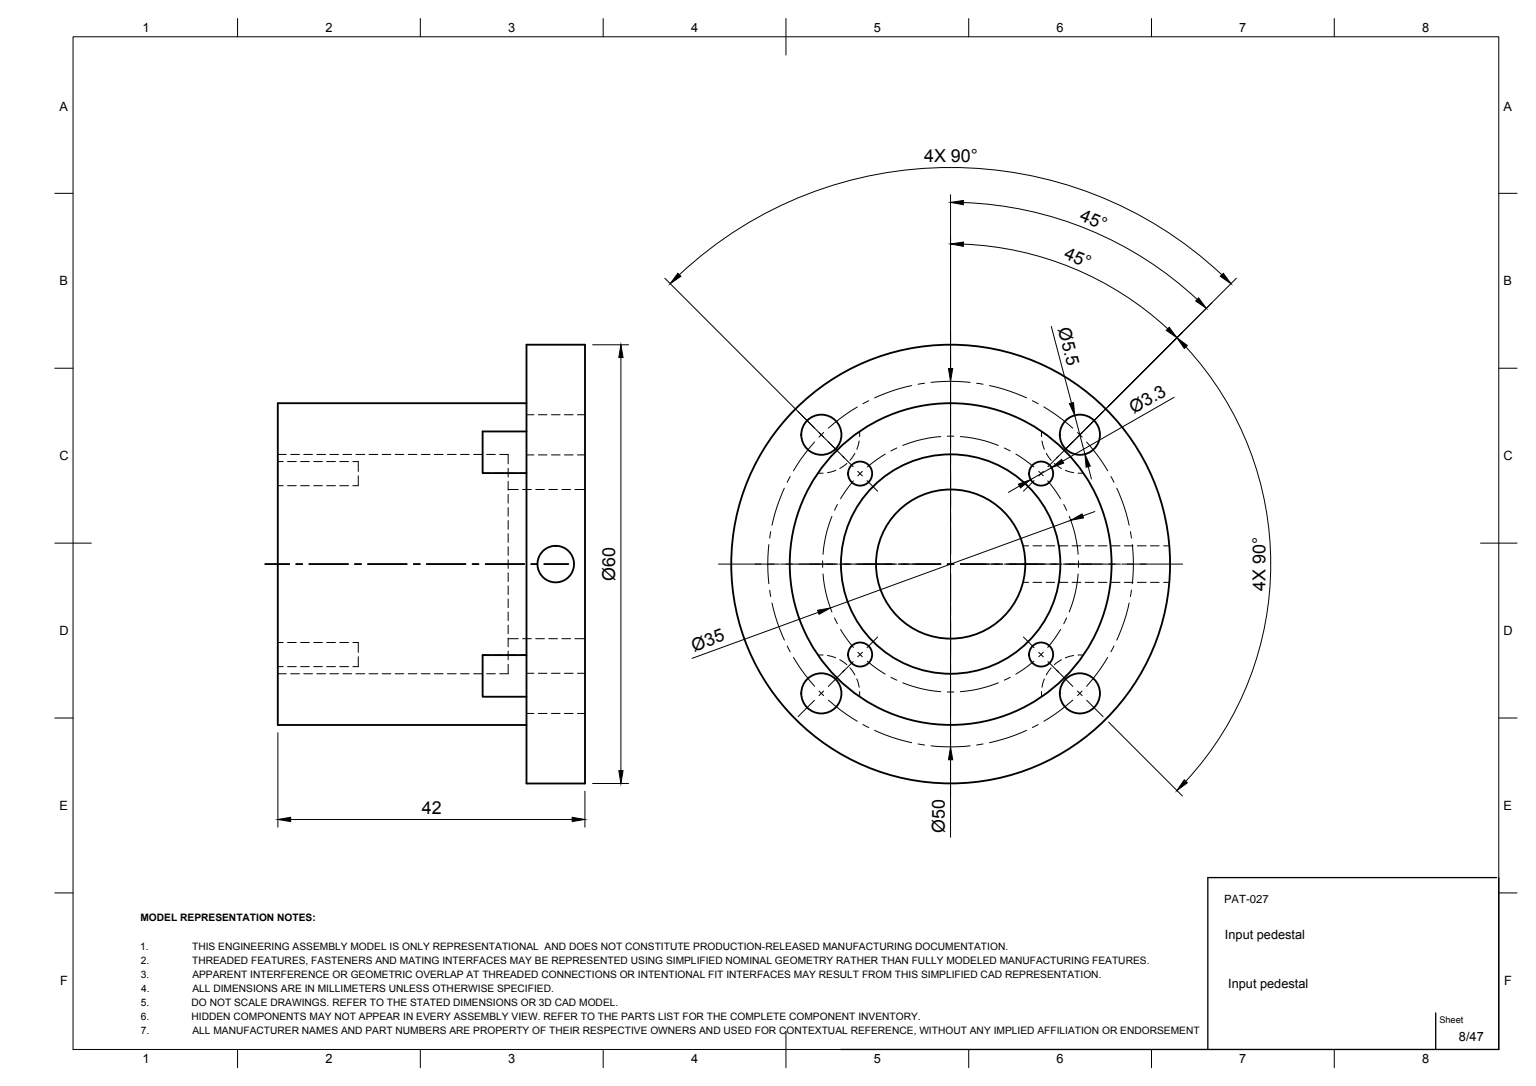
ISO-10303-21;
HEADER;
/* Generated by software containing ST-Developer
 * from STEP Tools, Inc. (www.steptools.com) 
 */

FILE_DESCRIPTION(
/* description */ ('Crank-driven oscillating fan base (mechanism only)'),

/* implementation_level */ '2;1');

FILE_NAME(
/* name */ 'Input pedestal.step',
/* time_stamp */ '2026-10-28T03:25:00-07:00',
/* author */ (''),
/* organization */ (''),
/* preprocessor_version */ 'ST-DEVELOPER v20.2',
/* originating_system */ 'Autodesk Translation Framework v15.17.0.0',
/* authorisation */ '');

FILE_SCHEMA (('AUTOMOTIVE_DESIGN { 1 0 10303 214 3 1 1 }'));
ENDSEC;

DATA;
#10=MECHANICAL_DESIGN_GEOMETRIC_PRESENTATION_REPRESENTATION('',(#440),#11916);
#316=B_SPLINE_CURVE_WITH_KNOTS('',3,(#9676,#9677,#9678,#9679,#9680,#9681,
#9682,#9683,#9684,#9685),.UNSPECIFIED.,.F.,.F.,(4,2,2,2,4),(0.,0.0945941824764479,
0.189188364952896,0.283770357603024,0.378352350253152),.UNSPECIFIED.);
#317=B_SPLINE_CURVE_WITH_KNOTS('',3,(#9686,#9687,#9688,#9689,#9690,#9691,
#9692,#9693,#9694,#9695,#9696,#9697,#9698,#9699,#9700,#9701,#9702,#9703,
#9704,#9705,#9706,#9707,#9708,#9709,#9710,#9711),.UNSPECIFIED.,.F.,.F.,
(4,2,2,2,2,2,2,2,2,2,2,2,4),(0.378352350253152,0.47293434290328,0.567516335553408,
0.662110518029855,0.756704700506303,0.851298882982751,0.945893065459199,
1.04047505810933,1.13505705075946,1.22963904340958,1.32422103605971,1.41881521853616,
1.51340940101261),.UNSPECIFIED.);
#318=B_SPLINE_CURVE_WITH_KNOTS('',3,(#9715,#9716,#9717,#9718,#9719,#9720,
#9721,#9722,#9723,#9724,#9725,#9726,#9727,#9728,#9729,#9730,#9731,#9732,
#9733,#9734,#9735,#9736,#9737,#9738,#9739,#9740),.UNSPECIFIED.,.F.,.F.,
(4,2,2,2,2,2,2,2,2,2,2,2,4),(0.,0.0942186410044058,0.188437282008812,0.282655768798837,
0.376874255588861,0.471092742378886,0.565311229168911,0.659529870173317,
0.753748511177723,0.847967152182129,0.942185793186535,1.03640427997656,
1.13062276676658),.UNSPECIFIED.);
#319=B_SPLINE_CURVE_WITH_KNOTS('',3,(#9741,#9742,#9743,#9744,#9745,#9746,
#9747,#9748,#9749,#9750),.UNSPECIFIED.,.F.,.F.,(4,2,2,2,4),(1.13062276676658,
1.22484125355661,1.31905974034663,1.41327838135104,1.50749702235545),
 .UNSPECIFIED.);
#360=SHAPE_REPRESENTATION_RELATIONSHIP('SRR','None',#12084,#400);
#400=ADVANCED_BREP_SHAPE_REPRESENTATION('',(#488),#11875);
#440=STYLED_ITEM('',(#12389),#488);
#488=MANIFOLD_SOLID_BREP('Body1',#6070);
#546=FACE_BOUND('',#1313,.T.);
#547=FACE_BOUND('',#1314,.T.);
#548=FACE_BOUND('',#1315,.T.);
#549=FACE_BOUND('',#1316,.T.);
#550=FACE_BOUND('',#1317,.T.);
#551=FACE_BOUND('',#1333,.T.);
#552=FACE_BOUND('',#1335,.T.);
#553=FACE_BOUND('',#1337,.T.);
#554=FACE_BOUND('',#1339,.T.);
#555=FACE_BOUND('',#1340,.T.);
#556=FACE_BOUND('',#1341,.T.);
#557=FACE_BOUND('',#1342,.T.);
#558=FACE_BOUND('',#1343,.T.);
#559=FACE_BOUND('',#1345,.T.);
#560=FACE_BOUND('',#1346,.T.);
#561=FACE_BOUND('',#1347,.T.);
#562=FACE_BOUND('',#1348,.T.);
#563=FACE_BOUND('',#1349,.T.);
#710=PLANE('',#6607);
#711=PLANE('',#6615);
#712=PLANE('',#6620);
#713=PLANE('',#6625);
#714=PLANE('',#6634);
#715=PLANE('',#6643);
#716=PLANE('',#6647);
#717=PLANE('',#6651);
#718=PLANE('',#6655);
#719=PLANE('',#6668);
#720=PLANE('',#6674);
#721=PLANE('',#6675);
#912=FACE_OUTER_BOUND('',#1303,.T.);
#913=FACE_OUTER_BOUND('',#1304,.T.);
#914=FACE_OUTER_BOUND('',#1305,.T.);
#915=FACE_OUTER_BOUND('',#1306,.T.);
#916=FACE_OUTER_BOUND('',#1307,.T.);
#917=FACE_OUTER_BOUND('',#1308,.T.);
#918=FACE_OUTER_BOUND('',#1309,.T.);
#919=FACE_OUTER_BOUND('',#1310,.T.);
#920=FACE_OUTER_BOUND('',#1311,.T.);
#921=FACE_OUTER_BOUND('',#1312,.T.);
#922=FACE_OUTER_BOUND('',#1318,.T.);
#923=FACE_OUTER_BOUND('',#1319,.T.);
#924=FACE_OUTER_BOUND('',#1320,.T.);
#925=FACE_OUTER_BOUND('',#1321,.T.);
#926=FACE_OUTER_BOUND('',#1322,.T.);
#927=FACE_OUTER_BOUND('',#1323,.T.);
#928=FACE_OUTER_BOUND('',#1324,.T.);
#929=FACE_OUTER_BOUND('',#1325,.T.);
#930=FACE_OUTER_BOUND('',#1326,.T.);
#931=FACE_OUTER_BOUND('',#1327,.T.);
#932=FACE_OUTER_BOUND('',#1328,.T.);
#933=FACE_OUTER_BOUND('',#1329,.T.);
#934=FACE_OUTER_BOUND('',#1330,.T.);
#935=FACE_OUTER_BOUND('',#1331,.T.);
#936=FACE_OUTER_BOUND('',#1332,.T.);
#937=FACE_OUTER_BOUND('',#1334,.T.);
#938=FACE_OUTER_BOUND('',#1336,.T.);
#939=FACE_OUTER_BOUND('',#1338,.T.);
#940=FACE_OUTER_BOUND('',#1344,.T.);
#1303=EDGE_LOOP('',(#4188,#4189));
#1304=EDGE_LOOP('',(#4190,#4191,#4192,#4193));
#1305=EDGE_LOOP('',(#4194,#4195,#4196,#4197));
#1306=EDGE_LOOP('',(#4198,#4199));
#1307=EDGE_LOOP('',(#4200,#4201,#4202,#4203));
#1308=EDGE_LOOP('',(#4204,#4205));
#1309=EDGE_LOOP('',(#4206,#4207,#4208,#4209));
#1310=EDGE_LOOP('',(#4210,#4211));
#1311=EDGE_LOOP('',(#4212,#4213,#4214,#4215,#4216,#4217,#4218,#4219,#4220,
#4221,#4222,#4223,#4224,#4225,#4226,#4227,#4228,#4229,#4230,#4231));
#1312=EDGE_LOOP('',(#4232));
#1313=EDGE_LOOP('',(#4233,#4234,#4235,#4236,#4237,#4238,#4239,#4240,#4241));
#1314=EDGE_LOOP('',(#4242));
#1315=EDGE_LOOP('',(#4243));
#1316=EDGE_LOOP('',(#4244));
#1317=EDGE_LOOP('',(#4245));
#1318=EDGE_LOOP('',(#4246,#4247,#4248,#4249));
#1319=EDGE_LOOP('',(#4250));
#1320=EDGE_LOOP('',(#4251,#4252,#4253,#4254));
#1321=EDGE_LOOP('',(#4255));
#1322=EDGE_LOOP('',(#4256,#4257,#4258,#4259));
#1323=EDGE_LOOP('',(#4260));
#1324=EDGE_LOOP('',(#4261,#4262,#4263,#4264));
#1325=EDGE_LOOP('',(#4265));
#1326=EDGE_LOOP('',(#4266,#4267,#4268,#4269,#4270,#4271));
#1327=EDGE_LOOP('',(#4272,#4273,#4274,#4275));
#1328=EDGE_LOOP('',(#4276,#4277,#4278,#4279));
#1329=EDGE_LOOP('',(#4280,#4281,#4282,#4283));
#1330=EDGE_LOOP('',(#4284,#4285,#4286,#4287));
#1331=EDGE_LOOP('',(#4288,#4289,#4290,#4291));
#1332=EDGE_LOOP('',(#4292));
#1333=EDGE_LOOP('',(#4293));
#1334=EDGE_LOOP('',(#4294,#4295,#4296,#4297));
#1335=EDGE_LOOP('',(#4298,#4299));
#1336=EDGE_LOOP('',(#4300,#4301,#4302,#4303));
#1337=EDGE_LOOP('',(#4304,#4305));
#1338=EDGE_LOOP('',(#4306));
#1339=EDGE_LOOP('',(#4307));
#1340=EDGE_LOOP('',(#4308));
#1341=EDGE_LOOP('',(#4309));
#1342=EDGE_LOOP('',(#4310));
#1343=EDGE_LOOP('',(#4311));
#1344=EDGE_LOOP('',(#4312));
#1345=EDGE_LOOP('',(#4313));
#1346=EDGE_LOOP('',(#4314));
#1347=EDGE_LOOP('',(#4315));
#1348=EDGE_LOOP('',(#4316));
#1349=EDGE_LOOP('',(#4317));
#1842=LINE('',#9587,#2175);
#1843=LINE('',#9590,#2176);
#1844=LINE('',#9594,#2177);
#1845=LINE('',#9598,#2178);
#1846=LINE('',#9605,#2179);
#1847=LINE('',#9609,#2180);
#1848=LINE('',#9616,#2181);
#1849=LINE('',#9620,#2182);
#1850=LINE('',#9628,#2183);
#1851=LINE('',#9649,#2184);
#1852=LINE('',#9656,#2185);
#1853=LINE('',#9663,#2186);
#1854=LINE('',#9670,#2187);
#1855=LINE('',#9713,#2188);
#1856=LINE('',#9754,#2189);
#1857=LINE('',#9758,#2190);
#1858=LINE('',#9762,#2191);
#1859=LINE('',#9766,#2192);
#1860=LINE('',#9771,#2193);
#1861=LINE('',#9778,#2194);
#1862=LINE('',#9782,#2195);
#2175=VECTOR('',#7559,1.);
#2176=VECTOR('',#7562,1.);
#2177=VECTOR('',#7565,1.);
#2178=VECTOR('',#7568,1.);
#2179=VECTOR('',#7577,1.);
#2180=VECTOR('',#7580,1.);
#2181=VECTOR('',#7589,1.);
#2182=VECTOR('',#7592,1.);
#2183=VECTOR('',#7603,2.2);
#2184=VECTOR('',#7630,0.165);
#2185=VECTOR('',#7639,0.165);
#2186=VECTOR('',#7648,0.165);
#2187=VECTOR('',#7657,0.165);
#2188=VECTOR('',#7664,0.25);
#2189=VECTOR('',#7669,0.275);
#2190=VECTOR('',#7674,0.275);
#2191=VECTOR('',#7679,0.275);
#2192=VECTOR('',#7684,0.275);
#2193=VECTOR('',#7689,1.5);
#2194=VECTOR('',#7698,3.);
#2195=VECTOR('',#7703,1.02);
#2480=CIRCLE('',#6608,2.2);
#2481=CIRCLE('',#6609,0.525);
#2482=CIRCLE('',#6611,0.525);
#2483=CIRCLE('',#6613,0.525);
#2484=CIRCLE('',#6614,0.525);
#2485=CIRCLE('',#6616,2.2);
#2486=CIRCLE('',#6618,0.525);
#2487=CIRCLE('',#6619,0.525);
#2488=CIRCLE('',#6621,2.2);
#2489=CIRCLE('',#6623,0.525);
#2490=CIRCLE('',#6624,0.525);
#2491=CIRCLE('',#6626,2.2);
#2492=CIRCLE('',#6628,2.2);
#2493=CIRCLE('',#6629,2.2);
#2494=CIRCLE('',#6630,2.2);
#2495=CIRCLE('',#6631,2.2);
#2496=CIRCLE('',#6632,2.2);
#2497=CIRCLE('',#6633,2.2);
#2498=CIRCLE('',#6635,3.);
#2499=CIRCLE('',#6636,0.275);
#2500=CIRCLE('',#6637,0.275);
#2501=CIRCLE('',#6638,0.275);
#2502=CIRCLE('',#6639,0.275);
#2503=CIRCLE('',#6641,0.165);
#2504=CIRCLE('',#6642,0.165);
#2505=CIRCLE('',#6645,0.165);
#2506=CIRCLE('',#6646,0.165);
#2507=CIRCLE('',#6649,0.165);
#2508=CIRCLE('',#6650,0.165);
#2509=CIRCLE('',#6653,0.165);
#2510=CIRCLE('',#6654,0.165);
#2511=CIRCLE('',#6658,0.275);
#2512=CIRCLE('',#6660,0.275);
#2513=CIRCLE('',#6662,0.275);
#2514=CIRCLE('',#6664,0.275);
#2515=CIRCLE('',#6666,1.5);
#2516=CIRCLE('',#6667,1.5);
#2517=CIRCLE('',#6669,1.02);
#2518=CIRCLE('',#6671,3.);
#2519=CIRCLE('',#6673,1.02);
#2869=VERTEX_POINT('',#9581);
#2870=VERTEX_POINT('',#9582);
#2871=VERTEX_POINT('',#9586);
#2872=VERTEX_POINT('',#9588);
#2873=VERTEX_POINT('',#9592);
#2874=VERTEX_POINT('',#9593);
#2875=VERTEX_POINT('',#9595);
#2876=VERTEX_POINT('',#9597);
#2877=VERTEX_POINT('',#9603);
#2878=VERTEX_POINT('',#9604);
#2879=VERTEX_POINT('',#9606);
#2880=VERTEX_POINT('',#9608);
#2881=VERTEX_POINT('',#9614);
#2882=VERTEX_POINT('',#9615);
#2883=VERTEX_POINT('',#9617);
#2884=VERTEX_POINT('',#9619);
#2885=VERTEX_POINT('',#9625);
#2886=VERTEX_POINT('',#9627);
#2887=VERTEX_POINT('',#9635);
#2888=VERTEX_POINT('',#9637);
#2889=VERTEX_POINT('',#9639);
#2890=VERTEX_POINT('',#9641);
#2891=VERTEX_POINT('',#9643);
#2892=VERTEX_POINT('',#9646);
#2893=VERTEX_POINT('',#9648);
#2894=VERTEX_POINT('',#9653);
#2895=VERTEX_POINT('',#9655);
#2896=VERTEX_POINT('',#9660);
#2897=VERTEX_POINT('',#9662);
#2898=VERTEX_POINT('',#9667);
#2899=VERTEX_POINT('',#9669);
#2900=VERTEX_POINT('',#9674);
#2901=VERTEX_POINT('',#9675);
#2902=VERTEX_POINT('',#9712);
#2903=VERTEX_POINT('',#9714);
#2904=VERTEX_POINT('',#9752);
#2905=VERTEX_POINT('',#9756);
#2906=VERTEX_POINT('',#9760);
#2907=VERTEX_POINT('',#9764);
#2908=VERTEX_POINT('',#9768);
#2909=VERTEX_POINT('',#9770);
#2910=VERTEX_POINT('',#9774);
#2911=VERTEX_POINT('',#9777);
#2912=VERTEX_POINT('',#9781);
#3389=EDGE_CURVE('',#2869,#2870,#2480,.T.);
#3390=EDGE_CURVE('',#2870,#2869,#2481,.T.);
#3391=EDGE_CURVE('',#2871,#2869,#1842,.T.);
#3392=EDGE_CURVE('',#2872,#2871,#2482,.T.);
#3393=EDGE_CURVE('',#2870,#2872,#1843,.T.);
#3394=EDGE_CURVE('',#2873,#2874,#1844,.T.);
#3395=EDGE_CURVE('',#2873,#2875,#2483,.T.);
#3396=EDGE_CURVE('',#2876,#2875,#1845,.T.);
#3397=EDGE_CURVE('',#2874,#2876,#2484,.T.);
#3398=EDGE_CURVE('',#2875,#2873,#2485,.T.);
#3399=EDGE_CURVE('',#2877,#2878,#1846,.T.);
#3400=EDGE_CURVE('',#2877,#2879,#2486,.T.);
#3401=EDGE_CURVE('',#2880,#2879,#1847,.T.);
#3402=EDGE_CURVE('',#2878,#2880,#2487,.T.);
#3403=EDGE_CURVE('',#2879,#2877,#2488,.T.);
#3404=EDGE_CURVE('',#2881,#2882,#1848,.T.);
#3405=EDGE_CURVE('',#2881,#2883,#2489,.T.);
#3406=EDGE_CURVE('',#2884,#2883,#1849,.T.);
#3407=EDGE_CURVE('',#2882,#2884,#2490,.T.);
#3408=EDGE_CURVE('',#2883,#2881,#2491,.T.);
#3409=EDGE_CURVE('',#2885,#2885,#2492,.T.);
#3410=EDGE_CURVE('',#2885,#2886,#1850,.T.);
#3411=EDGE_CURVE('',#2886,#2871,#2493,.T.);
#3412=EDGE_CURVE('',#2872,#2884,#2494,.T.);
#3413=EDGE_CURVE('',#2882,#2880,#2495,.T.);
#3414=EDGE_CURVE('',#2878,#2876,#2496,.T.);
#3415=EDGE_CURVE('',#2874,#2886,#2497,.T.);
#3416=EDGE_CURVE('',#2887,#2887,#2498,.T.);
#3417=EDGE_CURVE('',#2888,#2888,#2499,.T.);
#3418=EDGE_CURVE('',#2889,#2889,#2500,.T.);
#3419=EDGE_CURVE('',#2890,#2890,#2501,.T.);
#3420=EDGE_CURVE('',#2891,#2891,#2502,.T.);
#3421=EDGE_CURVE('',#2892,#2892,#2503,.T.);
#3422=EDGE_CURVE('',#2892,#2893,#1851,.T.);
#3423=EDGE_CURVE('',#2893,#2893,#2504,.T.);
#3424=EDGE_CURVE('',#2894,#2894,#2505,.T.);
#3425=EDGE_CURVE('',#2894,#2895,#1852,.T.);
#3426=EDGE_CURVE('',#2895,#2895,#2506,.T.);
#3427=EDGE_CURVE('',#2896,#2896,#2507,.T.);
#3428=EDGE_CURVE('',#2896,#2897,#1853,.T.);
#3429=EDGE_CURVE('',#2897,#2897,#2508,.T.);
#3430=EDGE_CURVE('',#2898,#2898,#2509,.T.);
#3431=EDGE_CURVE('',#2898,#2899,#1854,.T.);
#3432=EDGE_CURVE('',#2899,#2899,#2510,.T.);
#3433=EDGE_CURVE('',#2900,#2901,#316,.T.);
#3434=EDGE_CURVE('',#2901,#2900,#317,.T.);
#3435=EDGE_CURVE('',#2901,#2902,#1855,.T.);
#3436=EDGE_CURVE('',#2903,#2902,#318,.T.);
#3437=EDGE_CURVE('',#2902,#2903,#319,.T.);
#3438=EDGE_CURVE('',#2904,#2904,#2511,.T.);
#3439=EDGE_CURVE('',#2904,#2888,#1856,.T.);
#3440=EDGE_CURVE('',#2905,#2905,#2512,.T.);
#3441=EDGE_CURVE('',#2905,#2891,#1857,.T.);
#3442=EDGE_CURVE('',#2906,#2906,#2513,.T.);
#3443=EDGE_CURVE('',#2906,#2889,#1858,.T.);
#3444=EDGE_CURVE('',#2907,#2907,#2514,.T.);
#3445=EDGE_CURVE('',#2907,#2890,#1859,.T.);
#3446=EDGE_CURVE('',#2908,#2908,#2515,.T.);
#3447=EDGE_CURVE('',#2908,#2909,#1860,.T.);
#3448=EDGE_CURVE('',#2909,#2909,#2516,.T.);
#3449=EDGE_CURVE('',#2910,#2910,#2517,.T.);
#3450=EDGE_CURVE('',#2887,#2911,#1861,.T.);
#3451=EDGE_CURVE('',#2911,#2911,#2518,.T.);
#3452=EDGE_CURVE('',#2910,#2912,#1862,.T.);
#3453=EDGE_CURVE('',#2912,#2912,#2519,.T.);
#4188=ORIENTED_EDGE('',*,*,#3389,.F.);
#4189=ORIENTED_EDGE('',*,*,#3390,.F.);
#4190=ORIENTED_EDGE('',*,*,#3391,.F.);
#4191=ORIENTED_EDGE('',*,*,#3392,.F.);
#4192=ORIENTED_EDGE('',*,*,#3393,.F.);
#4193=ORIENTED_EDGE('',*,*,#3390,.T.);
#4194=ORIENTED_EDGE('',*,*,#3394,.F.);
#4195=ORIENTED_EDGE('',*,*,#3395,.T.);
#4196=ORIENTED_EDGE('',*,*,#3396,.F.);
#4197=ORIENTED_EDGE('',*,*,#3397,.F.);
#4198=ORIENTED_EDGE('',*,*,#3398,.F.);
#4199=ORIENTED_EDGE('',*,*,#3395,.F.);
#4200=ORIENTED_EDGE('',*,*,#3399,.F.);
#4201=ORIENTED_EDGE('',*,*,#3400,.T.);
#4202=ORIENTED_EDGE('',*,*,#3401,.F.);
#4203=ORIENTED_EDGE('',*,*,#3402,.F.);
#4204=ORIENTED_EDGE('',*,*,#3403,.F.);
#4205=ORIENTED_EDGE('',*,*,#3400,.F.);
#4206=ORIENTED_EDGE('',*,*,#3404,.F.);
#4207=ORIENTED_EDGE('',*,*,#3405,.T.);
#4208=ORIENTED_EDGE('',*,*,#3406,.F.);
#4209=ORIENTED_EDGE('',*,*,#3407,.F.);
#4210=ORIENTED_EDGE('',*,*,#3408,.F.);
#4211=ORIENTED_EDGE('',*,*,#3405,.F.);
#4212=ORIENTED_EDGE('',*,*,#3409,.F.);
#4213=ORIENTED_EDGE('',*,*,#3410,.T.);
#4214=ORIENTED_EDGE('',*,*,#3411,.T.);
#4215=ORIENTED_EDGE('',*,*,#3391,.T.);
#4216=ORIENTED_EDGE('',*,*,#3389,.T.);
#4217=ORIENTED_EDGE('',*,*,#3393,.T.);
#4218=ORIENTED_EDGE('',*,*,#3412,.T.);
#4219=ORIENTED_EDGE('',*,*,#3406,.T.);
#4220=ORIENTED_EDGE('',*,*,#3408,.T.);
#4221=ORIENTED_EDGE('',*,*,#3404,.T.);
#4222=ORIENTED_EDGE('',*,*,#3413,.T.);
#4223=ORIENTED_EDGE('',*,*,#3401,.T.);
#4224=ORIENTED_EDGE('',*,*,#3403,.T.);
#4225=ORIENTED_EDGE('',*,*,#3399,.T.);
#4226=ORIENTED_EDGE('',*,*,#3414,.T.);
#4227=ORIENTED_EDGE('',*,*,#3396,.T.);
#4228=ORIENTED_EDGE('',*,*,#3398,.T.);
#4229=ORIENTED_EDGE('',*,*,#3394,.T.);
#4230=ORIENTED_EDGE('',*,*,#3415,.T.);
#4231=ORIENTED_EDGE('',*,*,#3410,.F.);
#4232=ORIENTED_EDGE('',*,*,#3416,.T.);
#4233=ORIENTED_EDGE('',*,*,#3415,.F.);
#4234=ORIENTED_EDGE('',*,*,#3397,.T.);
#4235=ORIENTED_EDGE('',*,*,#3414,.F.);
#4236=ORIENTED_EDGE('',*,*,#3402,.T.);
#4237=ORIENTED_EDGE('',*,*,#3413,.F.);
#4238=ORIENTED_EDGE('',*,*,#3407,.T.);
#4239=ORIENTED_EDGE('',*,*,#3412,.F.);
#4240=ORIENTED_EDGE('',*,*,#3392,.T.);
#4241=ORIENTED_EDGE('',*,*,#3411,.F.);
#4242=ORIENTED_EDGE('',*,*,#3417,.T.);
#4243=ORIENTED_EDGE('',*,*,#3418,.T.);
#4244=ORIENTED_EDGE('',*,*,#3419,.T.);
#4245=ORIENTED_EDGE('',*,*,#3420,.T.);
#4246=ORIENTED_EDGE('',*,*,#3421,.F.);
#4247=ORIENTED_EDGE('',*,*,#3422,.T.);
#4248=ORIENTED_EDGE('',*,*,#3423,.F.);
#4249=ORIENTED_EDGE('',*,*,#3422,.F.);
#4250=ORIENTED_EDGE('',*,*,#3421,.T.);
#4251=ORIENTED_EDGE('',*,*,#3424,.F.);
#4252=ORIENTED_EDGE('',*,*,#3425,.T.);
#4253=ORIENTED_EDGE('',*,*,#3426,.F.);
#4254=ORIENTED_EDGE('',*,*,#3425,.F.);
#4255=ORIENTED_EDGE('',*,*,#3424,.T.);
#4256=ORIENTED_EDGE('',*,*,#3427,.F.);
#4257=ORIENTED_EDGE('',*,*,#3428,.T.);
#4258=ORIENTED_EDGE('',*,*,#3429,.F.);
#4259=ORIENTED_EDGE('',*,*,#3428,.F.);
#4260=ORIENTED_EDGE('',*,*,#3427,.T.);
#4261=ORIENTED_EDGE('',*,*,#3430,.F.);
#4262=ORIENTED_EDGE('',*,*,#3431,.T.);
#4263=ORIENTED_EDGE('',*,*,#3432,.F.);
#4264=ORIENTED_EDGE('',*,*,#3431,.F.);
#4265=ORIENTED_EDGE('',*,*,#3430,.T.);
#4266=ORIENTED_EDGE('',*,*,#3433,.F.);
#4267=ORIENTED_EDGE('',*,*,#3434,.F.);
#4268=ORIENTED_EDGE('',*,*,#3435,.T.);
#4269=ORIENTED_EDGE('',*,*,#3436,.F.);
#4270=ORIENTED_EDGE('',*,*,#3437,.F.);
#4271=ORIENTED_EDGE('',*,*,#3435,.F.);
#4272=ORIENTED_EDGE('',*,*,#3438,.F.);
#4273=ORIENTED_EDGE('',*,*,#3439,.T.);
#4274=ORIENTED_EDGE('',*,*,#3417,.F.);
#4275=ORIENTED_EDGE('',*,*,#3439,.F.);
#4276=ORIENTED_EDGE('',*,*,#3440,.F.);
#4277=ORIENTED_EDGE('',*,*,#3441,.T.);
#4278=ORIENTED_EDGE('',*,*,#3420,.F.);
#4279=ORIENTED_EDGE('',*,*,#3441,.F.);
#4280=ORIENTED_EDGE('',*,*,#3442,.F.);
#4281=ORIENTED_EDGE('',*,*,#3443,.T.);
#4282=ORIENTED_EDGE('',*,*,#3418,.F.);
#4283=ORIENTED_EDGE('',*,*,#3443,.F.);
#4284=ORIENTED_EDGE('',*,*,#3444,.F.);
#4285=ORIENTED_EDGE('',*,*,#3445,.T.);
#4286=ORIENTED_EDGE('',*,*,#3419,.F.);
#4287=ORIENTED_EDGE('',*,*,#3445,.F.);
#4288=ORIENTED_EDGE('',*,*,#3446,.F.);
#4289=ORIENTED_EDGE('',*,*,#3447,.T.);
#4290=ORIENTED_EDGE('',*,*,#3448,.F.);
#4291=ORIENTED_EDGE('',*,*,#3447,.F.);
#4292=ORIENTED_EDGE('',*,*,#3446,.T.);
#4293=ORIENTED_EDGE('',*,*,#3449,.F.);
#4294=ORIENTED_EDGE('',*,*,#3416,.F.);
#4295=ORIENTED_EDGE('',*,*,#3450,.T.);
#4296=ORIENTED_EDGE('',*,*,#3451,.T.);
#4297=ORIENTED_EDGE('',*,*,#3450,.F.);
#4298=ORIENTED_EDGE('',*,*,#3436,.T.);
#4299=ORIENTED_EDGE('',*,*,#3437,.T.);
#4300=ORIENTED_EDGE('',*,*,#3449,.T.);
#4301=ORIENTED_EDGE('',*,*,#3452,.T.);
#4302=ORIENTED_EDGE('',*,*,#3453,.T.);
#4303=ORIENTED_EDGE('',*,*,#3452,.F.);
#4304=ORIENTED_EDGE('',*,*,#3433,.T.);
#4305=ORIENTED_EDGE('',*,*,#3434,.T.);
#4306=ORIENTED_EDGE('',*,*,#3409,.T.);
#4307=ORIENTED_EDGE('',*,*,#3448,.T.);
#4308=ORIENTED_EDGE('',*,*,#3432,.T.);
#4309=ORIENTED_EDGE('',*,*,#3429,.T.);
#4310=ORIENTED_EDGE('',*,*,#3426,.T.);
#4311=ORIENTED_EDGE('',*,*,#3423,.T.);
#4312=ORIENTED_EDGE('',*,*,#3451,.F.);
#4313=ORIENTED_EDGE('',*,*,#3453,.F.);
#4314=ORIENTED_EDGE('',*,*,#3444,.T.);
#4315=ORIENTED_EDGE('',*,*,#3442,.T.);
#4316=ORIENTED_EDGE('',*,*,#3440,.T.);
#4317=ORIENTED_EDGE('',*,*,#3438,.T.);
#5554=CYLINDRICAL_SURFACE('',#6610,0.525);
#5555=CYLINDRICAL_SURFACE('',#6612,0.525);
#5556=CYLINDRICAL_SURFACE('',#6617,0.525);
#5557=CYLINDRICAL_SURFACE('',#6622,0.525);
#5558=CYLINDRICAL_SURFACE('',#6627,2.2);
#5559=CYLINDRICAL_SURFACE('',#6640,0.165);
#5560=CYLINDRICAL_SURFACE('',#6644,0.165);
#5561=CYLINDRICAL_SURFACE('',#6648,0.165);
#5562=CYLINDRICAL_SURFACE('',#6652,0.165);
#5563=CYLINDRICAL_SURFACE('',#6656,0.25);
#5564=CYLINDRICAL_SURFACE('',#6657,0.275);
#5565=CYLINDRICAL_SURFACE('',#6659,0.275);
#5566=CYLINDRICAL_SURFACE('',#6661,0.275);
#5567=CYLINDRICAL_SURFACE('',#6663,0.275);
#5568=CYLINDRICAL_SURFACE('',#6665,1.5);
#5569=CYLINDRICAL_SURFACE('',#6670,3.);
#5570=CYLINDRICAL_SURFACE('',#6672,1.02);
#5718=ADVANCED_FACE('',(#912),#710,.F.);
#5719=ADVANCED_FACE('',(#913),#5554,.F.);
#5720=ADVANCED_FACE('',(#914),#5555,.F.);
#5721=ADVANCED_FACE('',(#915),#711,.F.);
#5722=ADVANCED_FACE('',(#916),#5556,.F.);
#5723=ADVANCED_FACE('',(#917),#712,.F.);
#5724=ADVANCED_FACE('',(#918),#5557,.F.);
#5725=ADVANCED_FACE('',(#919),#713,.F.);
#5726=ADVANCED_FACE('',(#920),#5558,.T.);
#5727=ADVANCED_FACE('',(#921,#546,#547,#548,#549,#550),#714,.T.);
#5728=ADVANCED_FACE('',(#922),#5559,.F.);
#5729=ADVANCED_FACE('',(#923),#715,.T.);
#5730=ADVANCED_FACE('',(#924),#5560,.F.);
#5731=ADVANCED_FACE('',(#925),#716,.T.);
#5732=ADVANCED_FACE('',(#926),#5561,.F.);
#5733=ADVANCED_FACE('',(#927),#717,.T.);
#5734=ADVANCED_FACE('',(#928),#5562,.F.);
#5735=ADVANCED_FACE('',(#929),#718,.T.);
#5736=ADVANCED_FACE('',(#930),#5563,.F.);
#5737=ADVANCED_FACE('',(#931),#5564,.F.);
#5738=ADVANCED_FACE('',(#932),#5565,.F.);
#5739=ADVANCED_FACE('',(#933),#5566,.F.);
#5740=ADVANCED_FACE('',(#934),#5567,.F.);
#5741=ADVANCED_FACE('',(#935),#5568,.F.);
#5742=ADVANCED_FACE('',(#936,#551),#719,.T.);
#5743=ADVANCED_FACE('',(#937,#552),#5569,.T.);
#5744=ADVANCED_FACE('',(#938,#553),#5570,.F.);
#5745=ADVANCED_FACE('',(#939,#554,#555,#556,#557,#558),#720,.T.);
#5746=ADVANCED_FACE('',(#940,#559,#560,#561,#562,#563),#721,.F.);
#6070=CLOSED_SHELL('',(#5718,#5719,#5720,#5721,#5722,#5723,#5724,#5725,
#5726,#5727,#5728,#5729,#5730,#5731,#5732,#5733,#5734,#5735,#5736,#5737,
#5738,#5739,#5740,#5741,#5742,#5743,#5744,#5745,#5746));
#6606=AXIS2_PLACEMENT_3D('',#9579,#7549,#7550);
#6607=AXIS2_PLACEMENT_3D('',#9580,#7551,#7552);
#6608=AXIS2_PLACEMENT_3D('',#9583,#7553,#7554);
#6609=AXIS2_PLACEMENT_3D('',#9584,#7555,#7556);
#6610=AXIS2_PLACEMENT_3D('',#9585,#7557,#7558);
#6611=AXIS2_PLACEMENT_3D('',#9589,#7560,#7561);
#6612=AXIS2_PLACEMENT_3D('',#9591,#7563,#7564);
#6613=AXIS2_PLACEMENT_3D('',#9596,#7566,#7567);
#6614=AXIS2_PLACEMENT_3D('',#9599,#7569,#7570);
#6615=AXIS2_PLACEMENT_3D('',#9600,#7571,#7572);
#6616=AXIS2_PLACEMENT_3D('',#9601,#7573,#7574);
#6617=AXIS2_PLACEMENT_3D('',#9602,#7575,#7576);
#6618=AXIS2_PLACEMENT_3D('',#9607,#7578,#7579);
#6619=AXIS2_PLACEMENT_3D('',#9610,#7581,#7582);
#6620=AXIS2_PLACEMENT_3D('',#9611,#7583,#7584);
#6621=AXIS2_PLACEMENT_3D('',#9612,#7585,#7586);
#6622=AXIS2_PLACEMENT_3D('',#9613,#7587,#7588);
#6623=AXIS2_PLACEMENT_3D('',#9618,#7590,#7591);
#6624=AXIS2_PLACEMENT_3D('',#9621,#7593,#7594);
#6625=AXIS2_PLACEMENT_3D('',#9622,#7595,#7596);
#6626=AXIS2_PLACEMENT_3D('',#9623,#7597,#7598);
#6627=AXIS2_PLACEMENT_3D('',#9624,#7599,#7600);
#6628=AXIS2_PLACEMENT_3D('',#9626,#7601,#7602);
#6629=AXIS2_PLACEMENT_3D('',#9629,#7604,#7605);
#6630=AXIS2_PLACEMENT_3D('',#9630,#7606,#7607);
#6631=AXIS2_PLACEMENT_3D('',#9631,#7608,#7609);
#6632=AXIS2_PLACEMENT_3D('',#9632,#7610,#7611);
#6633=AXIS2_PLACEMENT_3D('',#9633,#7612,#7613);
#6634=AXIS2_PLACEMENT_3D('',#9634,#7614,#7615);
#6635=AXIS2_PLACEMENT_3D('',#9636,#7616,#7617);
#6636=AXIS2_PLACEMENT_3D('',#9638,#7618,#7619);
#6637=AXIS2_PLACEMENT_3D('',#9640,#7620,#7621);
#6638=AXIS2_PLACEMENT_3D('',#9642,#7622,#7623);
#6639=AXIS2_PLACEMENT_3D('',#9644,#7624,#7625);
#6640=AXIS2_PLACEMENT_3D('',#9645,#7626,#7627);
#6641=AXIS2_PLACEMENT_3D('',#9647,#7628,#7629);
#6642=AXIS2_PLACEMENT_3D('',#9650,#7631,#7632);
#6643=AXIS2_PLACEMENT_3D('',#9651,#7633,#7634);
#6644=AXIS2_PLACEMENT_3D('',#9652,#7635,#7636);
#6645=AXIS2_PLACEMENT_3D('',#9654,#7637,#7638);
#6646=AXIS2_PLACEMENT_3D('',#9657,#7640,#7641);
#6647=AXIS2_PLACEMENT_3D('',#9658,#7642,#7643);
#6648=AXIS2_PLACEMENT_3D('',#9659,#7644,#7645);
#6649=AXIS2_PLACEMENT_3D('',#9661,#7646,#7647);
#6650=AXIS2_PLACEMENT_3D('',#9664,#7649,#7650);
#6651=AXIS2_PLACEMENT_3D('',#9665,#7651,#7652);
#6652=AXIS2_PLACEMENT_3D('',#9666,#7653,#7654);
#6653=AXIS2_PLACEMENT_3D('',#9668,#7655,#7656);
#6654=AXIS2_PLACEMENT_3D('',#9671,#7658,#7659);
#6655=AXIS2_PLACEMENT_3D('',#9672,#7660,#7661);
#6656=AXIS2_PLACEMENT_3D('',#9673,#7662,#7663);
#6657=AXIS2_PLACEMENT_3D('',#9751,#7665,#7666);
#6658=AXIS2_PLACEMENT_3D('',#9753,#7667,#7668);
#6659=AXIS2_PLACEMENT_3D('',#9755,#7670,#7671);
#6660=AXIS2_PLACEMENT_3D('',#9757,#7672,#7673);
#6661=AXIS2_PLACEMENT_3D('',#9759,#7675,#7676);
#6662=AXIS2_PLACEMENT_3D('',#9761,#7677,#7678);
#6663=AXIS2_PLACEMENT_3D('',#9763,#7680,#7681);
#6664=AXIS2_PLACEMENT_3D('',#9765,#7682,#7683);
#6665=AXIS2_PLACEMENT_3D('',#9767,#7685,#7686);
#6666=AXIS2_PLACEMENT_3D('',#9769,#7687,#7688);
#6667=AXIS2_PLACEMENT_3D('',#9772,#7690,#7691);
#6668=AXIS2_PLACEMENT_3D('',#9773,#7692,#7693);
#6669=AXIS2_PLACEMENT_3D('',#9775,#7694,#7695);
#6670=AXIS2_PLACEMENT_3D('',#9776,#7696,#7697);
#6671=AXIS2_PLACEMENT_3D('',#9779,#7699,#7700);
#6672=AXIS2_PLACEMENT_3D('',#9780,#7701,#7702);
#6673=AXIS2_PLACEMENT_3D('',#9783,#7704,#7705);
#6674=AXIS2_PLACEMENT_3D('',#9784,#7706,#7707);
#6675=AXIS2_PLACEMENT_3D('',#9785,#7708,#7709);
#7549=DIRECTION('axis',(0.,0.,1.));
#7550=DIRECTION('refdir',(1.,0.,0.));
#7551=DIRECTION('center_axis',(0.,0.,1.));
#7552=DIRECTION('ref_axis',(1.,0.,0.));
#7553=DIRECTION('center_axis',(0.,0.,1.));
#7554=DIRECTION('ref_axis',(1.,0.,0.));
#7555=DIRECTION('center_axis',(0.,0.,1.));
#7556=DIRECTION('ref_axis',(1.,0.,0.));
#7557=DIRECTION('center_axis',(0.,0.,1.));
#7558=DIRECTION('ref_axis',(1.,0.,0.));
#7559=DIRECTION('',(0.,0.,1.));
#7560=DIRECTION('center_axis',(0.,0.,1.));
#7561=DIRECTION('ref_axis',(1.,0.,0.));
#7562=DIRECTION('',(0.,0.,-1.));
#7563=DIRECTION('center_axis',(0.,0.,1.));
#7564=DIRECTION('ref_axis',(1.,0.,0.));
#7565=DIRECTION('',(0.,0.,-1.));
#7566=DIRECTION('center_axis',(0.,0.,1.));
#7567=DIRECTION('ref_axis',(1.,0.,0.));
#7568=DIRECTION('',(0.,0.,1.));
#7569=DIRECTION('center_axis',(0.,0.,1.));
#7570=DIRECTION('ref_axis',(1.,0.,0.));
#7571=DIRECTION('center_axis',(0.,0.,1.));
#7572=DIRECTION('ref_axis',(1.,0.,0.));
#7573=DIRECTION('center_axis',(0.,0.,1.));
#7574=DIRECTION('ref_axis',(1.,0.,0.));
#7575=DIRECTION('center_axis',(0.,0.,1.));
#7576=DIRECTION('ref_axis',(-0.707106781186548,-0.707106781186547,0.));
#7577=DIRECTION('',(0.,0.,-1.));
#7578=DIRECTION('center_axis',(0.,0.,1.));
#7579=DIRECTION('ref_axis',(1.,0.,0.));
#7580=DIRECTION('',(0.,0.,1.));
#7581=DIRECTION('center_axis',(0.,0.,1.));
#7582=DIRECTION('ref_axis',(1.,0.,0.));
#7583=DIRECTION('center_axis',(0.,0.,1.));
#7584=DIRECTION('ref_axis',(1.,0.,0.));
#7585=DIRECTION('center_axis',(0.,0.,1.));
#7586=DIRECTION('ref_axis',(1.,0.,0.));
#7587=DIRECTION('center_axis',(0.,0.,1.));
#7588=DIRECTION('ref_axis',(-0.707106781186547,0.707106781186548,0.));
#7589=DIRECTION('',(0.,0.,-1.));
#7590=DIRECTION('center_axis',(0.,0.,1.));
#7591=DIRECTION('ref_axis',(1.,0.,0.));
#7592=DIRECTION('',(0.,0.,1.));
#7593=DIRECTION('center_axis',(0.,0.,1.));
#7594=DIRECTION('ref_axis',(1.,0.,0.));
#7595=DIRECTION('center_axis',(0.,0.,1.));
#7596=DIRECTION('ref_axis',(1.,0.,0.));
#7597=DIRECTION('center_axis',(0.,0.,1.));
#7598=DIRECTION('ref_axis',(1.,0.,0.));
#7599=DIRECTION('center_axis',(0.,0.,1.));
#7600=DIRECTION('ref_axis',(1.,0.,0.));
#7601=DIRECTION('center_axis',(0.,0.,1.));
#7602=DIRECTION('ref_axis',(1.,0.,0.));
#7603=DIRECTION('',(0.,0.,-1.));
#7604=DIRECTION('center_axis',(0.,0.,1.));
#7605=DIRECTION('ref_axis',(1.,0.,0.));
#7606=DIRECTION('center_axis',(0.,0.,1.));
#7607=DIRECTION('ref_axis',(1.,0.,0.));
#7608=DIRECTION('center_axis',(0.,0.,1.));
#7609=DIRECTION('ref_axis',(1.,0.,0.));
#7610=DIRECTION('center_axis',(0.,0.,1.));
#7611=DIRECTION('ref_axis',(1.,0.,0.));
#7612=DIRECTION('center_axis',(0.,0.,1.));
#7613=DIRECTION('ref_axis',(1.,0.,0.));
#7614=DIRECTION('center_axis',(0.,0.,1.));
#7615=DIRECTION('ref_axis',(1.,0.,0.));
#7616=DIRECTION('center_axis',(0.,0.,1.));
#7617=DIRECTION('ref_axis',(1.,0.,0.));
#7618=DIRECTION('center_axis',(0.,0.,-1.));
#7619=DIRECTION('ref_axis',(1.,0.,0.));
#7620=DIRECTION('center_axis',(0.,0.,-1.));
#7621=DIRECTION('ref_axis',(1.,0.,0.));
#7622=DIRECTION('center_axis',(0.,0.,-1.));
#7623=DIRECTION('ref_axis',(1.,0.,0.));
#7624=DIRECTION('center_axis',(0.,0.,-1.));
#7625=DIRECTION('ref_axis',(1.,0.,0.));
#7626=DIRECTION('center_axis',(0.,0.,1.));
#7627=DIRECTION('ref_axis',(1.,0.,0.));
#7628=DIRECTION('center_axis',(0.,0.,1.));
#7629=DIRECTION('ref_axis',(1.,0.,0.));
#7630=DIRECTION('',(0.,0.,1.));
#7631=DIRECTION('center_axis',(0.,0.,-1.));
#7632=DIRECTION('ref_axis',(1.,0.,0.));
#7633=DIRECTION('center_axis',(0.,0.,1.));
#7634=DIRECTION('ref_axis',(1.,0.,0.));
#7635=DIRECTION('center_axis',(0.,0.,1.));
#7636=DIRECTION('ref_axis',(1.,0.,0.));
#7637=DIRECTION('center_axis',(0.,0.,1.));
#7638=DIRECTION('ref_axis',(1.,0.,0.));
#7639=DIRECTION('',(0.,0.,1.));
#7640=DIRECTION('center_axis',(0.,0.,-1.));
#7641=DIRECTION('ref_axis',(1.,0.,0.));
#7642=DIRECTION('center_axis',(0.,0.,1.));
#7643=DIRECTION('ref_axis',(1.,0.,0.));
#7644=DIRECTION('center_axis',(0.,0.,1.));
#7645=DIRECTION('ref_axis',(1.,0.,0.));
#7646=DIRECTION('center_axis',(0.,0.,1.));
#7647=DIRECTION('ref_axis',(1.,0.,0.));
#7648=DIRECTION('',(0.,0.,1.));
#7649=DIRECTION('center_axis',(0.,0.,-1.));
#7650=DIRECTION('ref_axis',(1.,0.,0.));
#7651=DIRECTION('center_axis',(0.,0.,1.));
#7652=DIRECTION('ref_axis',(1.,0.,0.));
#7653=DIRECTION('center_axis',(0.,0.,1.));
#7654=DIRECTION('ref_axis',(1.,0.,0.));
#7655=DIRECTION('center_axis',(0.,0.,1.));
#7656=DIRECTION('ref_axis',(1.,0.,0.));
#7657=DIRECTION('',(0.,0.,1.));
#7658=DIRECTION('center_axis',(0.,0.,-1.));
#7659=DIRECTION('ref_axis',(1.,0.,0.));
#7660=DIRECTION('center_axis',(0.,0.,1.));
#7661=DIRECTION('ref_axis',(1.,0.,0.));
#7662=DIRECTION('center_axis',(1.,0.,0.));
#7663=DIRECTION('ref_axis',(0.,0.,-1.));
#7664=DIRECTION('',(1.,0.,0.));
#7665=DIRECTION('center_axis',(0.,0.,1.));
#7666=DIRECTION('ref_axis',(1.,0.,0.));
#7667=DIRECTION('center_axis',(0.,0.,1.));
#7668=DIRECTION('ref_axis',(1.,0.,0.));
#7669=DIRECTION('',(0.,0.,1.));
#7670=DIRECTION('center_axis',(0.,0.,1.));
#7671=DIRECTION('ref_axis',(1.,0.,0.));
#7672=DIRECTION('center_axis',(0.,0.,1.));
#7673=DIRECTION('ref_axis',(1.,0.,0.));
#7674=DIRECTION('',(0.,0.,1.));
#7675=DIRECTION('center_axis',(0.,0.,1.));
#7676=DIRECTION('ref_axis',(1.,0.,0.));
#7677=DIRECTION('center_axis',(0.,0.,1.));
#7678=DIRECTION('ref_axis',(1.,0.,0.));
#7679=DIRECTION('',(0.,0.,1.));
#7680=DIRECTION('center_axis',(0.,0.,1.));
#7681=DIRECTION('ref_axis',(1.,0.,0.));
#7682=DIRECTION('center_axis',(0.,0.,1.));
#7683=DIRECTION('ref_axis',(1.,0.,0.));
#7684=DIRECTION('',(0.,0.,1.));
#7685=DIRECTION('center_axis',(0.,0.,1.));
#7686=DIRECTION('ref_axis',(1.,0.,0.));
#7687=DIRECTION('center_axis',(0.,0.,1.));
#7688=DIRECTION('ref_axis',(1.,0.,0.));
#7689=DIRECTION('',(0.,0.,1.));
#7690=DIRECTION('center_axis',(0.,0.,-1.));
#7691=DIRECTION('ref_axis',(1.,0.,0.));
#7692=DIRECTION('center_axis',(0.,0.,1.));
#7693=DIRECTION('ref_axis',(1.,0.,0.));
#7694=DIRECTION('center_axis',(0.,0.,1.));
#7695=DIRECTION('ref_axis',(1.,0.,0.));
#7696=DIRECTION('center_axis',(0.,0.,1.));
#7697=DIRECTION('ref_axis',(1.,0.,0.));
#7698=DIRECTION('',(0.,0.,-1.));
#7699=DIRECTION('center_axis',(0.,0.,1.));
#7700=DIRECTION('ref_axis',(1.,0.,0.));
#7701=DIRECTION('center_axis',(0.,0.,1.));
#7702=DIRECTION('ref_axis',(1.,0.,0.));
#7703=DIRECTION('',(0.,0.,-1.));
#7704=DIRECTION('center_axis',(0.,0.,-1.));
#7705=DIRECTION('ref_axis',(1.,0.,0.));
#7706=DIRECTION('center_axis',(0.,0.,1.));
#7707=DIRECTION('ref_axis',(1.,0.,0.));
#7708=DIRECTION('center_axis',(0.,0.,1.));
#7709=DIRECTION('ref_axis',(1.,0.,0.));
#9579=CARTESIAN_POINT('',(0.,0.,0.));
#9580=CARTESIAN_POINT('Origin',(-1.76776695296637,-1.76776695296637,2.4));
#9581=CARTESIAN_POINT('',(-1.8139637388702,-1.24480341984751,2.4));
#9582=CARTESIAN_POINT('',(-1.24480341984751,-1.81396373887019,2.4));
#9583=CARTESIAN_POINT('Origin',(0.,0.,2.4));
#9584=CARTESIAN_POINT('Origin',(-1.76776695296637,-1.76776695296637,2.4));
#9585=CARTESIAN_POINT('Origin',(-1.76776695296637,-1.76776695296637,1.8));
#9586=CARTESIAN_POINT('',(-1.8139637388702,-1.24480341984751,1.8));
#9587=CARTESIAN_POINT('',(-1.8139637388702,-1.24480341984751,1.8));
#9588=CARTESIAN_POINT('',(-1.24480341984751,-1.81396373887019,1.8));
#9589=CARTESIAN_POINT('Origin',(-1.76776695296637,-1.76776695296637,1.8));
#9590=CARTESIAN_POINT('',(-1.24480341984751,-1.81396373887019,1.8));
#9591=CARTESIAN_POINT('Origin',(-1.76776695296637,1.76776695296637,1.8));
#9592=CARTESIAN_POINT('',(-1.81396373887019,1.24480341984751,2.4));
#9593=CARTESIAN_POINT('',(-1.81396373887019,1.24480341984751,1.8));
#9594=CARTESIAN_POINT('',(-1.81396373887019,1.24480341984751,1.8));
#9595=CARTESIAN_POINT('',(-1.24480341984751,1.81396373887019,2.4));
#9596=CARTESIAN_POINT('Origin',(-1.76776695296637,1.76776695296637,2.4));
#9597=CARTESIAN_POINT('',(-1.24480341984751,1.81396373887019,1.8));
#9598=CARTESIAN_POINT('',(-1.24480341984751,1.81396373887019,1.8));
#9599=CARTESIAN_POINT('Origin',(-1.76776695296637,1.76776695296637,1.8));
#9600=CARTESIAN_POINT('Origin',(-1.76776695296637,1.76776695296637,2.4));
#9601=CARTESIAN_POINT('Origin',(0.,0.,2.4));
#9602=CARTESIAN_POINT('Origin',(1.76776695296637,1.76776695296637,1.8));
#9603=CARTESIAN_POINT('',(1.24480341984751,1.81396373887019,2.4));
#9604=CARTESIAN_POINT('',(1.24480341984751,1.81396373887019,1.8));
#9605=CARTESIAN_POINT('',(1.24480341984751,1.81396373887019,1.8));
#9606=CARTESIAN_POINT('',(1.81396373887019,1.24480341984751,2.4));
#9607=CARTESIAN_POINT('Origin',(1.76776695296637,1.76776695296637,2.4));
#9608=CARTESIAN_POINT('',(1.81396373887019,1.24480341984751,1.8));
#9609=CARTESIAN_POINT('',(1.81396373887019,1.24480341984751,1.8));
#9610=CARTESIAN_POINT('Origin',(1.76776695296637,1.76776695296637,1.8));
#9611=CARTESIAN_POINT('Origin',(1.76776695296637,1.76776695296637,2.4));
#9612=CARTESIAN_POINT('Origin',(0.,0.,2.4));
#9613=CARTESIAN_POINT('Origin',(1.76776695296637,-1.76776695296637,1.8));
#9614=CARTESIAN_POINT('',(1.81396373887019,-1.24480341984751,2.4));
#9615=CARTESIAN_POINT('',(1.81396373887019,-1.24480341984751,1.8));
#9616=CARTESIAN_POINT('',(1.81396373887019,-1.24480341984751,1.8));
#9617=CARTESIAN_POINT('',(1.24480341984751,-1.8139637388702,2.4));
#9618=CARTESIAN_POINT('Origin',(1.76776695296637,-1.76776695296637,2.4));
#9619=CARTESIAN_POINT('',(1.24480341984751,-1.8139637388702,1.8));
#9620=CARTESIAN_POINT('',(1.24480341984751,-1.8139637388702,1.8));
#9621=CARTESIAN_POINT('Origin',(1.76776695296637,-1.76776695296637,1.8));
#9622=CARTESIAN_POINT('Origin',(1.76776695296637,-1.76776695296637,2.4));
#9623=CARTESIAN_POINT('Origin',(0.,0.,2.4));
#9624=CARTESIAN_POINT('Origin',(0.,0.,1.));
#9625=CARTESIAN_POINT('',(-2.2,-2.69422295812418E-16,5.2));
#9626=CARTESIAN_POINT('Origin',(0.,0.,5.2));
#9627=CARTESIAN_POINT('',(-2.2,-2.69422295812418E-16,1.8));
#9628=CARTESIAN_POINT('',(-2.2,-2.69422295812418E-16,1.));
#9629=CARTESIAN_POINT('Origin',(0.,0.,1.8));
#9630=CARTESIAN_POINT('Origin',(0.,0.,1.8));
#9631=CARTESIAN_POINT('Origin',(0.,0.,1.8));
#9632=CARTESIAN_POINT('Origin',(0.,0.,1.8));
#9633=CARTESIAN_POINT('Origin',(0.,0.,1.8));
#9634=CARTESIAN_POINT('Origin',(0.,0.,1.8));
#9635=CARTESIAN_POINT('',(-3.,-3.67394039744206E-16,1.8));
#9636=CARTESIAN_POINT('Origin',(0.,0.,1.8));
#9637=CARTESIAN_POINT('',(-2.04276695296637,-1.76776695296637,1.8));
#9638=CARTESIAN_POINT('Origin',(-1.76776695296637,-1.76776695296637,1.8));
#9639=CARTESIAN_POINT('',(1.49276695296637,1.76776695296637,1.8));
#9640=CARTESIAN_POINT('Origin',(1.76776695296637,1.76776695296637,1.8));
#9641=CARTESIAN_POINT('',(1.49276695296637,-1.76776695296637,1.8));
#9642=CARTESIAN_POINT('Origin',(1.76776695296637,-1.76776695296637,1.8));
#9643=CARTESIAN_POINT('',(-2.04276695296637,1.76776695296637,1.8));
#9644=CARTESIAN_POINT('Origin',(-1.76776695296637,1.76776695296637,1.8));
#9645=CARTESIAN_POINT('Origin',(-1.23743686707646,-1.23743686707646,4.1));
#9646=CARTESIAN_POINT('',(-1.40243686707646,-1.23743686707646,4.1));
#9647=CARTESIAN_POINT('Origin',(-1.23743686707646,-1.23743686707646,4.1));
#9648=CARTESIAN_POINT('',(-1.40243686707646,-1.23743686707646,5.2));
#9649=CARTESIAN_POINT('',(-1.40243686707646,-1.23743686707646,4.1));
#9650=CARTESIAN_POINT('Origin',(-1.23743686707646,-1.23743686707646,5.2));
#9651=CARTESIAN_POINT('Origin',(-1.23743686707646,-1.23743686707646,4.1));
#9652=CARTESIAN_POINT('Origin',(-1.23743686707646,1.23743686707646,4.1));
#9653=CARTESIAN_POINT('',(-1.40243686707646,1.23743686707646,4.1));
#9654=CARTESIAN_POINT('Origin',(-1.23743686707646,1.23743686707646,4.1));
#9655=CARTESIAN_POINT('',(-1.40243686707646,1.23743686707646,5.2));
#9656=CARTESIAN_POINT('',(-1.40243686707646,1.23743686707646,4.1));
#9657=CARTESIAN_POINT('Origin',(-1.23743686707646,1.23743686707646,5.2));
#9658=CARTESIAN_POINT('Origin',(-1.23743686707646,1.23743686707646,4.1));
#9659=CARTESIAN_POINT('Origin',(1.23743686707646,1.23743686707646,4.1));
#9660=CARTESIAN_POINT('',(1.07243686707646,1.23743686707646,4.1));
#9661=CARTESIAN_POINT('Origin',(1.23743686707646,1.23743686707646,4.1));
#9662=CARTESIAN_POINT('',(1.07243686707646,1.23743686707646,5.2));
#9663=CARTESIAN_POINT('',(1.07243686707646,1.23743686707646,4.1));
#9664=CARTESIAN_POINT('Origin',(1.23743686707646,1.23743686707646,5.2));
#9665=CARTESIAN_POINT('Origin',(1.23743686707646,1.23743686707646,4.1));
#9666=CARTESIAN_POINT('Origin',(1.23743686707646,-1.23743686707646,4.1));
#9667=CARTESIAN_POINT('',(1.07243686707646,-1.23743686707646,4.1));
#9668=CARTESIAN_POINT('Origin',(1.23743686707646,-1.23743686707646,4.1));
#9669=CARTESIAN_POINT('',(1.07243686707646,-1.23743686707646,5.2));
#9670=CARTESIAN_POINT('',(1.07243686707646,-1.23743686707646,4.1));
#9671=CARTESIAN_POINT('Origin',(1.23743686707646,-1.23743686707646,5.2));
#9672=CARTESIAN_POINT('Origin',(1.23743686707646,-1.23743686707646,4.1));
#9673=CARTESIAN_POINT('Origin',(0.9,0.,1.4));
#9674=CARTESIAN_POINT('',(0.988888264668966,0.25,1.4));
#9675=CARTESIAN_POINT('',(1.02,-1.18386380373883E-17,1.65));
#9676=CARTESIAN_POINT('Ctrl Pts',(0.988888264668966,0.25,1.4));
#9677=CARTESIAN_POINT('Ctrl Pts',(0.988888264668966,0.25,1.43153139415882));
#9678=CARTESIAN_POINT('Ctrl Pts',(0.990553370646674,0.243672048431404,1.46507214966317));
#9679=CARTESIAN_POINT('Ctrl Pts',(0.996491737296663,0.218119830014375,1.52662620974954));
#9680=CARTESIAN_POINT('Ctrl Pts',(1.00067109353237,0.198902128206072,1.5546512623872));
#9681=CARTESIAN_POINT('Ctrl Pts',(1.00845756932386,0.154654113568716,1.59889927702456));
#9682=CARTESIAN_POINT('Ctrl Pts',(1.01258144235289,0.126627870945253,1.61811920309393));
#9683=CARTESIAN_POINT('Ctrl Pts',(1.0183917429657,0.065069600391363,1.64367304400768));
#9684=CARTESIAN_POINT('Ctrl Pts',(1.02,0.031527330883376,1.65));
#9685=CARTESIAN_POINT('Ctrl Pts',(1.02,2.77555756156289E-17,1.65));
#9686=CARTESIAN_POINT('Ctrl Pts',(1.02,6.93889390390723E-18,1.65));
#9687=CARTESIAN_POINT('Ctrl Pts',(1.02,-0.031527330883376,1.65));
#9688=CARTESIAN_POINT('Ctrl Pts',(1.0183917429657,-0.065069600391363,1.64367304400768));
#9689=CARTESIAN_POINT('Ctrl Pts',(1.01258144235289,-0.126627870945253,1.61811920309393));
#9690=CARTESIAN_POINT('Ctrl Pts',(1.00845756932386,-0.154654113568716,1.59889927702456));
#9691=CARTESIAN_POINT('Ctrl Pts',(1.00067109353237,-0.198902128206072,1.5546512623872));
#9692=CARTESIAN_POINT('Ctrl Pts',(0.996491737296663,-0.218119830014375,
1.52662620974954));
#9693=CARTESIAN_POINT('Ctrl Pts',(0.990553370646674,-0.243672048431404,
1.46507214966317));
#9694=CARTESIAN_POINT('Ctrl Pts',(0.988888264668967,-0.25,1.43153139415882));
#9695=CARTESIAN_POINT('Ctrl Pts',(0.988888264668967,-0.25,1.36846860584118));
#9696=CARTESIAN_POINT('Ctrl Pts',(0.990553370646674,-0.243672048431404,
1.33492785033683));
#9697=CARTESIAN_POINT('Ctrl Pts',(0.996491737296663,-0.218119830014375,
1.27337379025046));
#9698=CARTESIAN_POINT('Ctrl Pts',(1.00067109353237,-0.198902128206072,1.2453487376128));
#9699=CARTESIAN_POINT('Ctrl Pts',(1.00845756932386,-0.154654113568716,1.20110072297544));
#9700=CARTESIAN_POINT('Ctrl Pts',(1.01258144235289,-0.126627870945254,1.18188079690607));
#9701=CARTESIAN_POINT('Ctrl Pts',(1.0183917429657,-0.0650696003913633,1.15632695599232));
#9702=CARTESIAN_POINT('Ctrl Pts',(1.02,-0.0315273308833761,1.15));
#9703=CARTESIAN_POINT('Ctrl Pts',(1.02,0.0315273308833759,1.15));
#9704=CARTESIAN_POINT('Ctrl Pts',(1.0183917429657,0.065069600391363,1.15632695599232));
#9705=CARTESIAN_POINT('Ctrl Pts',(1.01258144235289,0.126627870945253,1.18188079690607));
#9706=CARTESIAN_POINT('Ctrl Pts',(1.00845756932386,0.154654113568716,1.20110072297544));
#9707=CARTESIAN_POINT('Ctrl Pts',(1.00067109353237,0.198902128206072,1.2453487376128));
#9708=CARTESIAN_POINT('Ctrl Pts',(0.996491737296663,0.218119830014375,1.27337379025046));
#9709=CARTESIAN_POINT('Ctrl Pts',(0.990553370646674,0.243672048431404,1.33492785033683));
#9710=CARTESIAN_POINT('Ctrl Pts',(0.988888264668967,0.25,1.36846860584118));
#9711=CARTESIAN_POINT('Ctrl Pts',(0.988888264668967,0.25,1.4));
#9712=CARTESIAN_POINT('',(3.,-3.06161699786838E-17,1.65));
#9713=CARTESIAN_POINT('',(0.9,-3.06161699786838E-17,1.65));
#9714=CARTESIAN_POINT('',(2.98956518577535,0.25,1.4));
#9715=CARTESIAN_POINT('Ctrl Pts',(2.98956518577535,0.25,1.4));
#9716=CARTESIAN_POINT('Ctrl Pts',(2.98956518577535,0.25,1.36859378633186));
#9717=CARTESIAN_POINT('Ctrl Pts',(2.99011104995181,0.24372047740942,1.33510417960069));
#9718=CARTESIAN_POINT('Ctrl Pts',(2.99208145165098,0.218202539734559,1.27351367328886));
#9719=CARTESIAN_POINT('Ctrl Pts',(2.99347740802958,0.198964922639276,1.245411532046));
#9720=CARTESIAN_POINT('Ctrl Pts',(2.99609686518216,0.154588504271054,1.20103511367778));
#9721=CARTESIAN_POINT('Ctrl Pts',(2.99749070376198,0.126486346986081,1.18179746841036));
#9722=CARTESIAN_POINT('Ctrl Pts',(2.99945625936844,0.0648957875009219,1.15627950921557));
#9723=CARTESIAN_POINT('Ctrl Pts',(3.,0.0314061622633416,1.15));
#9724=CARTESIAN_POINT('Ctrl Pts',(3.,-0.0314061622633416,1.15));
#9725=CARTESIAN_POINT('Ctrl Pts',(2.99945625936844,-0.0648957875009221,
1.15627950921557));
#9726=CARTESIAN_POINT('Ctrl Pts',(2.99749070376198,-0.126486346986081,1.18179746841036));
#9727=CARTESIAN_POINT('Ctrl Pts',(2.99609686518216,-0.154588504271054,1.20103511367778));
#9728=CARTESIAN_POINT('Ctrl Pts',(2.99347740802958,-0.198964922639276,1.245411532046));
#9729=CARTESIAN_POINT('Ctrl Pts',(2.99208145165098,-0.218202539734559,1.27351367328886));
#9730=CARTESIAN_POINT('Ctrl Pts',(2.99011104995181,-0.24372047740942,1.33510417960069));
#9731=CARTESIAN_POINT('Ctrl Pts',(2.98956518577535,-0.25,1.36859378633186));
#9732=CARTESIAN_POINT('Ctrl Pts',(2.98956518577535,-0.25,1.43140621366814));
#9733=CARTESIAN_POINT('Ctrl Pts',(2.99011104995181,-0.24372047740942,1.4648958203993));
#9734=CARTESIAN_POINT('Ctrl Pts',(2.99208145165098,-0.21820253973456,1.52648632671114));
#9735=CARTESIAN_POINT('Ctrl Pts',(2.99347740802958,-0.198964922639276,1.554588467954));
#9736=CARTESIAN_POINT('Ctrl Pts',(2.99609686518216,-0.154588504271054,1.59896488632222));
#9737=CARTESIAN_POINT('Ctrl Pts',(2.99749070376198,-0.126486346986082,1.61820253158964));
#9738=CARTESIAN_POINT('Ctrl Pts',(2.99945625936844,-0.0648957875009221,
1.64372049078443));
#9739=CARTESIAN_POINT('Ctrl Pts',(3.,-0.0314061622633417,1.65));
#9740=CARTESIAN_POINT('Ctrl Pts',(3.,-5.55111512312578E-17,1.65));
#9741=CARTESIAN_POINT('Ctrl Pts',(3.,-2.08166817117217E-17,1.65));
#9742=CARTESIAN_POINT('Ctrl Pts',(3.,0.0314061622633416,1.65));
#9743=CARTESIAN_POINT('Ctrl Pts',(2.99945625936844,0.0648957875009221,1.64372049078443));
#9744=CARTESIAN_POINT('Ctrl Pts',(2.99749070376198,0.126486346986081,1.61820253158964));
#9745=CARTESIAN_POINT('Ctrl Pts',(2.99609686518216,0.154588504271054,1.59896488632222));
#9746=CARTESIAN_POINT('Ctrl Pts',(2.99347740802958,0.198964922639276,1.554588467954));
#9747=CARTESIAN_POINT('Ctrl Pts',(2.99208145165098,0.218202539734559,1.52648632671114));
#9748=CARTESIAN_POINT('Ctrl Pts',(2.99011104995181,0.24372047740942,1.46489582039931));
#9749=CARTESIAN_POINT('Ctrl Pts',(2.98956518577535,0.25,1.43140621366814));
#9750=CARTESIAN_POINT('Ctrl Pts',(2.98956518577535,0.25,1.4));
#9751=CARTESIAN_POINT('Origin',(-1.76776695296637,-1.76776695296637,0.9));
#9752=CARTESIAN_POINT('',(-2.04276695296637,-1.76776695296637,1.));
#9753=CARTESIAN_POINT('Origin',(-1.76776695296637,-1.76776695296637,1.));
#9754=CARTESIAN_POINT('',(-2.04276695296637,-1.76776695296637,0.9));
#9755=CARTESIAN_POINT('Origin',(-1.76776695296637,1.76776695296637,0.9));
#9756=CARTESIAN_POINT('',(-2.04276695296637,1.76776695296637,1.));
#9757=CARTESIAN_POINT('Origin',(-1.76776695296637,1.76776695296637,1.));
#9758=CARTESIAN_POINT('',(-2.04276695296637,1.76776695296637,0.9));
#9759=CARTESIAN_POINT('Origin',(1.76776695296637,1.76776695296637,0.9));
#9760=CARTESIAN_POINT('',(1.49276695296637,1.76776695296637,1.));
#9761=CARTESIAN_POINT('Origin',(1.76776695296637,1.76776695296637,1.));
#9762=CARTESIAN_POINT('',(1.49276695296637,1.76776695296637,0.9));
#9763=CARTESIAN_POINT('Origin',(1.76776695296637,-1.76776695296637,0.9));
#9764=CARTESIAN_POINT('',(1.49276695296637,-1.76776695296637,1.));
#9765=CARTESIAN_POINT('Origin',(1.76776695296637,-1.76776695296637,1.));
#9766=CARTESIAN_POINT('',(1.49276695296637,-1.76776695296637,0.9));
#9767=CARTESIAN_POINT('Origin',(0.,0.,2.05));
#9768=CARTESIAN_POINT('',(-1.5,-1.83697019872103E-16,2.05));
#9769=CARTESIAN_POINT('Origin',(0.,0.,2.05));
#9770=CARTESIAN_POINT('',(-1.5,1.83697019872103E-16,5.2));
#9771=CARTESIAN_POINT('',(-1.5,-1.83697019872103E-16,2.05));
#9772=CARTESIAN_POINT('Origin',(0.,0.,5.2));
#9773=CARTESIAN_POINT('Origin',(0.,0.,2.05));
#9774=CARTESIAN_POINT('',(-1.02,-1.2491397351303E-16,2.05));
#9775=CARTESIAN_POINT('Origin',(0.,0.,2.05));
#9776=CARTESIAN_POINT('Origin',(0.,0.,1.));
#9777=CARTESIAN_POINT('',(-3.,-3.67394039744206E-16,1.));
#9778=CARTESIAN_POINT('',(-3.,-3.67394039744206E-16,1.));
#9779=CARTESIAN_POINT('Origin',(0.,0.,1.));
#9780=CARTESIAN_POINT('Origin',(0.,0.,1.));
#9781=CARTESIAN_POINT('',(-1.02,-1.2491397351303E-16,1.));
#9782=CARTESIAN_POINT('',(-1.02,-1.2491397351303E-16,1.));
#9783=CARTESIAN_POINT('Origin',(0.,0.,1.));
#9784=CARTESIAN_POINT('Origin',(0.,0.,5.2));
#9785=CARTESIAN_POINT('Origin',(0.,0.,1.));
#11828=UNCERTAINTY_MEASURE_WITH_UNIT(LENGTH_MEASURE(0.001),#11917,
'DISTANCE_ACCURACY_VALUE',
'Maximum model space distance between geometric entities at asserted c
onnectivities');
#11869=UNCERTAINTY_MEASURE_WITH_UNIT(LENGTH_MEASURE(0.001),#11917,
'DISTANCE_ACCURACY_VALUE',
'Maximum model space distance between geometric entities at asserted c
onnectivities');
#11875=(
GEOMETRIC_REPRESENTATION_CONTEXT(3)
GLOBAL_UNCERTAINTY_ASSIGNED_CONTEXT((#11828))
GLOBAL_UNIT_ASSIGNED_CONTEXT((#11917,#11919,#11920))
REPRESENTATION_CONTEXT('','3D')
);
#11916=(
GEOMETRIC_REPRESENTATION_CONTEXT(3)
GLOBAL_UNCERTAINTY_ASSIGNED_CONTEXT((#11869))
GLOBAL_UNIT_ASSIGNED_CONTEXT((#11917,#11919,#11920))
REPRESENTATION_CONTEXT('','3D')
);
#11917=(
LENGTH_UNIT()
NAMED_UNIT(*)
SI_UNIT(.CENTI.,.METRE.)
);
#11919=(
NAMED_UNIT(*)
PLANE_ANGLE_UNIT()
SI_UNIT($,.RADIAN.)
);
#11920=(
NAMED_UNIT(*)
SI_UNIT($,.STERADIAN.)
SOLID_ANGLE_UNIT()
);
#11926=SHAPE_DEFINITION_REPRESENTATION(#11972,#12084);
#11972=PRODUCT_DEFINITION_SHAPE('',$,#12131);
#12084=SHAPE_REPRESENTATION('',(#6606),#11875);
#12125=PRODUCT_DEFINITION_CONTEXT('part definition',#12265,'design');
#12131=PRODUCT_DEFINITION('Input pedestal','Input pedestal',#12177,#12125);
#12177=PRODUCT_DEFINITION_FORMATION('',$,#12272);
#12265=APPLICATION_CONTEXT(
'Core Data for Automotive Mechanical Design Process');
#12266=PRODUCT_CONTEXT('part definition',#12265,'mechanical');
#12272=PRODUCT('Input pedestal','Input pedestal','Input pedestal',(#12266));
#12383=COLOUR_RGB('Off White',0.89,0.88,0.83);
#12384=FILL_AREA_STYLE_COLOUR('',#12383);
#12385=FILL_AREA_STYLE('',(#12384));
#12386=SURFACE_STYLE_FILL_AREA(#12385);
#12387=SURFACE_SIDE_STYLE('',(#12386));
#12388=SURFACE_STYLE_USAGE(.BOTH.,#12387);
#12389=PRESENTATION_STYLE_ASSIGNMENT((#12388));
ENDSEC;
END-ISO-10303-21;
